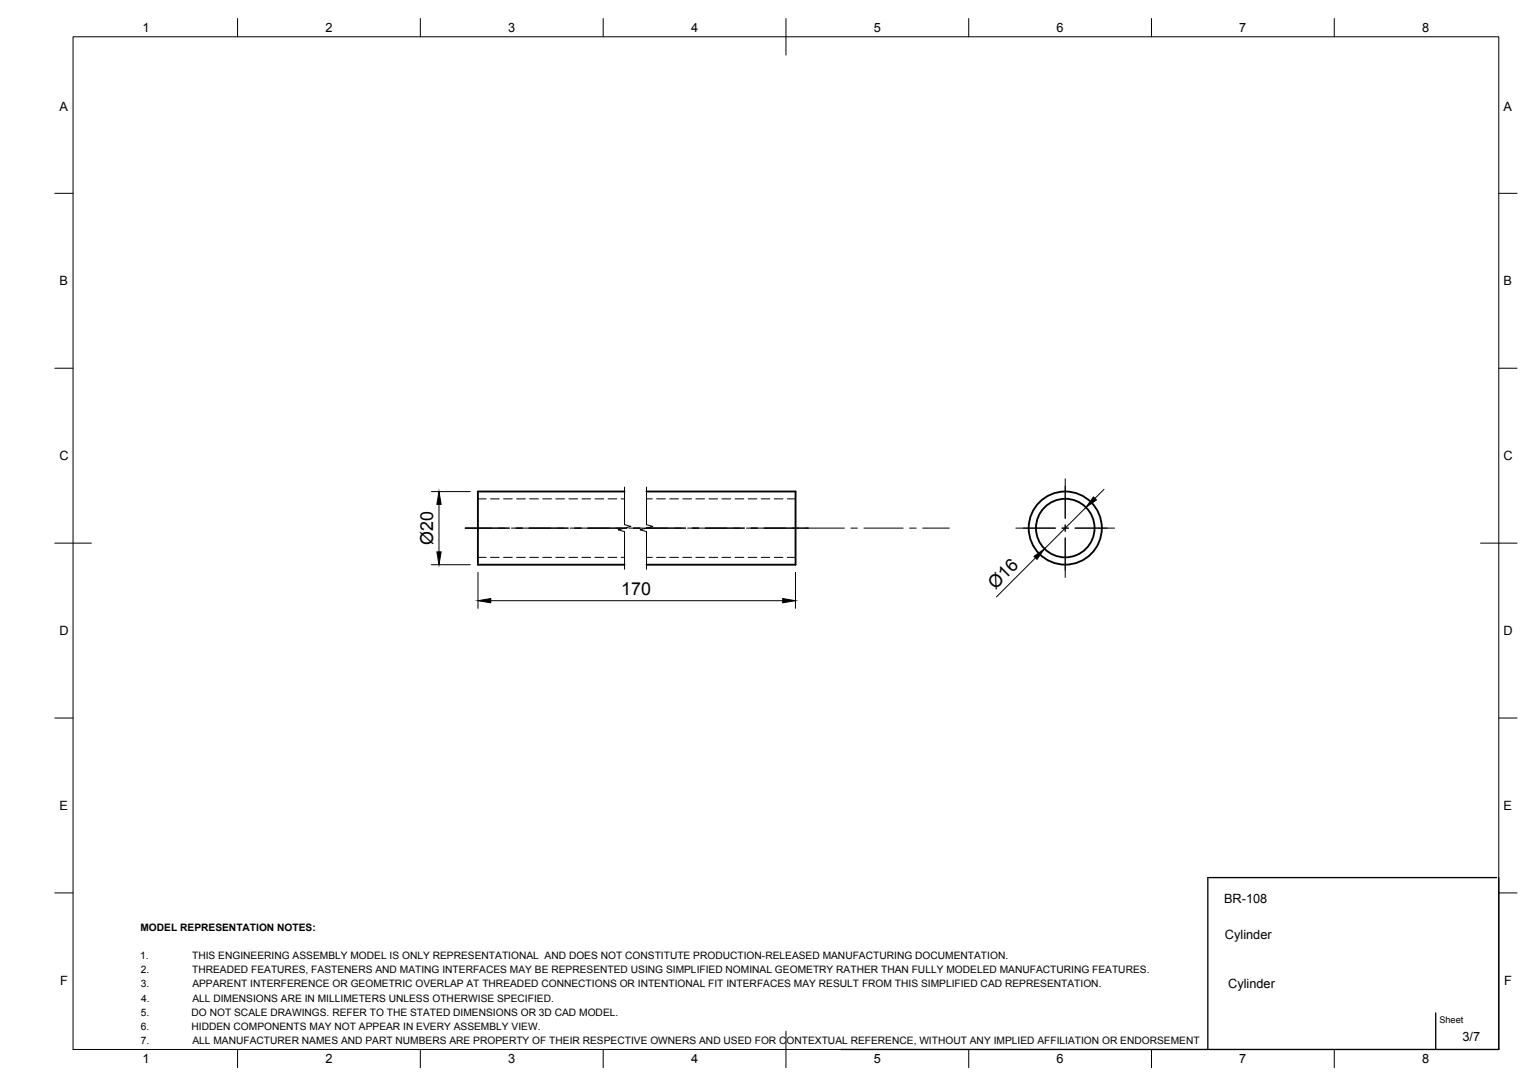
ISO-10303-21;
HEADER;
/* Generated by software containing ST-Developer
 * from STEP Tools, Inc. (www.steptools.com) 
 */

FILE_DESCRIPTION(
/* description */ (''),
/* implementation_level */ '2;1');

FILE_NAME(
/* name */ 'Cylinder.step',
/* time_stamp */ '2026-11-14T03:52:36-08:00',
/* author */ (''),
/* organization */ (''),
/* preprocessor_version */ 'ST-DEVELOPER v20.2',
/* originating_system */ 'Autodesk Translation Framework v15.17.0.0',
/* authorisation */ '');

FILE_SCHEMA (('AUTOMOTIVE_DESIGN { 1 0 10303 214 3 1 1 }'));
ENDSEC;

DATA;
#10=MECHANICAL_DESIGN_GEOMETRIC_PRESENTATION_REPRESENTATION('',(#191),#19443);
#175=SHAPE_REPRESENTATION_RELATIONSHIP('SRR','None',#19475,#183);
#183=ADVANCED_BREP_SHAPE_REPRESENTATION('',(#199),#19435);
#191=STYLED_ITEM('',(#19524),#199);
#199=MANIFOLD_SOLID_BREP('Body1',#2018);
#207=FACE_BOUND('',#372,.T.);
#208=FACE_BOUND('',#374,.T.);
#220=PLANE('',#2123);
#221=PLANE('',#2124);
#273=FACE_OUTER_BOUND('',#369,.T.);
#274=FACE_OUTER_BOUND('',#370,.T.);
#275=FACE_OUTER_BOUND('',#371,.T.);
#276=FACE_OUTER_BOUND('',#373,.T.);
#369=EDGE_LOOP('',(#1291,#1292,#1293,#1294));
#370=EDGE_LOOP('',(#1295,#1296,#1297,#1298));
#371=EDGE_LOOP('',(#1299));
#372=EDGE_LOOP('',(#1300));
#373=EDGE_LOOP('',(#1301));
#374=EDGE_LOOP('',(#1302));
#478=LINE('',#2701,#605);
#479=LINE('',#2707,#606);
#605=VECTOR('',#2274,8.);
#606=VECTOR('',#2281,10.);
#732=CIRCLE('',#2118,8.);
#733=CIRCLE('',#2119,8.);
#734=CIRCLE('',#2121,10.);
#735=CIRCLE('',#2122,10.);
#776=VERTEX_POINT('',#2698);
#777=VERTEX_POINT('',#2700);
#778=VERTEX_POINT('',#2704);
#779=VERTEX_POINT('',#2706);
#994=EDGE_CURVE('',#776,#776,#732,.T.);
#995=EDGE_CURVE('',#776,#777,#478,.T.);
#996=EDGE_CURVE('',#777,#777,#733,.T.);
#997=EDGE_CURVE('',#778,#778,#734,.T.);
#998=EDGE_CURVE('',#778,#779,#479,.T.);
#999=EDGE_CURVE('',#779,#779,#735,.T.);
#1291=ORIENTED_EDGE('',*,*,#994,.T.);
#1292=ORIENTED_EDGE('',*,*,#995,.T.);
#1293=ORIENTED_EDGE('',*,*,#996,.F.);
#1294=ORIENTED_EDGE('',*,*,#995,.F.);
#1295=ORIENTED_EDGE('',*,*,#997,.F.);
#1296=ORIENTED_EDGE('',*,*,#998,.T.);
#1297=ORIENTED_EDGE('',*,*,#999,.T.);
#1298=ORIENTED_EDGE('',*,*,#998,.F.);
#1299=ORIENTED_EDGE('',*,*,#997,.T.);
#1300=ORIENTED_EDGE('',*,*,#996,.T.);
#1301=ORIENTED_EDGE('',*,*,#999,.F.);
#1302=ORIENTED_EDGE('',*,*,#994,.F.);
#1885=CYLINDRICAL_SURFACE('',#2117,8.);
#1886=CYLINDRICAL_SURFACE('',#2120,10.);
#1922=ADVANCED_FACE('',(#273),#1885,.F.);
#1923=ADVANCED_FACE('',(#274),#1886,.T.);
#1924=ADVANCED_FACE('',(#275,#207),#220,.T.);
#1925=ADVANCED_FACE('',(#276,#208),#221,.F.);
#2018=CLOSED_SHELL('',(#1922,#1923,#1924,#1925));
#2116=AXIS2_PLACEMENT_3D('',#2696,#2268,#2269);
#2117=AXIS2_PLACEMENT_3D('',#2697,#2270,#2271);
#2118=AXIS2_PLACEMENT_3D('',#2699,#2272,#2273);
#2119=AXIS2_PLACEMENT_3D('',#2702,#2275,#2276);
#2120=AXIS2_PLACEMENT_3D('',#2703,#2277,#2278);
#2121=AXIS2_PLACEMENT_3D('',#2705,#2279,#2280);
#2122=AXIS2_PLACEMENT_3D('',#2708,#2282,#2283);
#2123=AXIS2_PLACEMENT_3D('',#2709,#2284,#2285);
#2124=AXIS2_PLACEMENT_3D('',#2710,#2286,#2287);
#2268=DIRECTION('axis',(0.,0.,1.));
#2269=DIRECTION('refdir',(1.,0.,0.));
#2270=DIRECTION('center_axis',(0.,0.,1.));
#2271=DIRECTION('ref_axis',(1.,0.,0.));
#2272=DIRECTION('center_axis',(0.,0.,-1.));
#2273=DIRECTION('ref_axis',(1.,0.,0.));
#2274=DIRECTION('',(0.,0.,1.));
#2275=DIRECTION('center_axis',(0.,0.,-1.));
#2276=DIRECTION('ref_axis',(1.,0.,0.));
#2277=DIRECTION('center_axis',(0.,0.,1.));
#2278=DIRECTION('ref_axis',(1.,0.,0.));
#2279=DIRECTION('center_axis',(0.,0.,1.));
#2280=DIRECTION('ref_axis',(1.,0.,0.));
#2281=DIRECTION('',(0.,0.,-1.));
#2282=DIRECTION('center_axis',(0.,0.,1.));
#2283=DIRECTION('ref_axis',(1.,0.,0.));
#2284=DIRECTION('center_axis',(0.,0.,1.));
#2285=DIRECTION('ref_axis',(1.,0.,0.));
#2286=DIRECTION('center_axis',(0.,0.,1.));
#2287=DIRECTION('ref_axis',(1.,0.,0.));
#2696=CARTESIAN_POINT('',(0.,0.,0.));
#2697=CARTESIAN_POINT('Origin',(0.,0.,0.));
#2698=CARTESIAN_POINT('',(-8.,-9.79717439317882E-16,0.));
#2699=CARTESIAN_POINT('Origin',(0.,0.,0.));
#2700=CARTESIAN_POINT('',(-8.,-9.79717439317882E-16,170.));
#2701=CARTESIAN_POINT('',(-8.,-9.79717439317883E-16,0.));
#2702=CARTESIAN_POINT('Origin',(0.,0.,170.));
#2703=CARTESIAN_POINT('Origin',(0.,0.,0.));
#2704=CARTESIAN_POINT('',(-10.,-1.22464679914735E-15,170.));
#2705=CARTESIAN_POINT('Origin',(0.,0.,170.));
#2706=CARTESIAN_POINT('',(-10.,-1.22464679914735E-15,0.));
#2707=CARTESIAN_POINT('',(-10.,-1.22464679914735E-15,0.));
#2708=CARTESIAN_POINT('Origin',(0.,0.,0.));
#2709=CARTESIAN_POINT('Origin',(0.,0.,170.));
#2710=CARTESIAN_POINT('Origin',(0.,0.,0.));
#19425=UNCERTAINTY_MEASURE_WITH_UNIT(LENGTH_MEASURE(0.01),#19444,
'DISTANCE_ACCURACY_VALUE',
'Maximum model space distance between geometric entities at asserted c
onnectivities');
#19433=UNCERTAINTY_MEASURE_WITH_UNIT(LENGTH_MEASURE(0.01),#19444,
'DISTANCE_ACCURACY_VALUE',
'Maximum model space distance between geometric entities at asserted c
onnectivities');
#19435=(
GEOMETRIC_REPRESENTATION_CONTEXT(3)
GLOBAL_UNCERTAINTY_ASSIGNED_CONTEXT((#19425))
GLOBAL_UNIT_ASSIGNED_CONTEXT((#19444,#19446,#19447))
REPRESENTATION_CONTEXT('','3D')
);
#19443=(
GEOMETRIC_REPRESENTATION_CONTEXT(3)
GLOBAL_UNCERTAINTY_ASSIGNED_CONTEXT((#19433))
GLOBAL_UNIT_ASSIGNED_CONTEXT((#19444,#19446,#19447))
REPRESENTATION_CONTEXT('','3D')
);
#19444=(
LENGTH_UNIT()
NAMED_UNIT(*)
SI_UNIT(.MILLI.,.METRE.)
);
#19446=(
NAMED_UNIT(*)
PLANE_ANGLE_UNIT()
SI_UNIT($,.RADIAN.)
);
#19447=(
NAMED_UNIT(*)
SI_UNIT($,.STERADIAN.)
SOLID_ANGLE_UNIT()
);
#19449=SHAPE_DEFINITION_REPRESENTATION(#19458,#19475);
#19458=PRODUCT_DEFINITION_SHAPE('',$,#19485);
#19475=SHAPE_REPRESENTATION('',(#2116),#19435);
#19483=PRODUCT_DEFINITION_CONTEXT('part definition',#19512,'design');
#19485=PRODUCT_DEFINITION('Cylinder','Cylinder',#19494,#19483);
#19494=PRODUCT_DEFINITION_FORMATION('',$,#19515);
#19512=APPLICATION_CONTEXT(
'Core Data for Automotive Mechanical Design Process');
#19513=PRODUCT_CONTEXT('part definition',#19512,'mechanical');
#19515=PRODUCT('Cylinder','Cylinder',$,(#19513));
#19524=PRESENTATION_STYLE_ASSIGNMENT((#19527));
#19527=SURFACE_STYLE_USAGE(.BOTH.,#19530);
#19530=SURFACE_SIDE_STYLE('',(#19533));
#19533=SURFACE_STYLE_FILL_AREA(#19536);
#19536=FILL_AREA_STYLE('Opaque(36,31,37)',(#19539));
#19539=FILL_AREA_STYLE_COLOUR('Opaque(36,31,37)',#19542);
#19542=COLOUR_RGB('Opaque(36,31,37)',0.141176470588235,0.12156862745098,
0.145098039215686);
ENDSEC;
END-ISO-10303-21;
